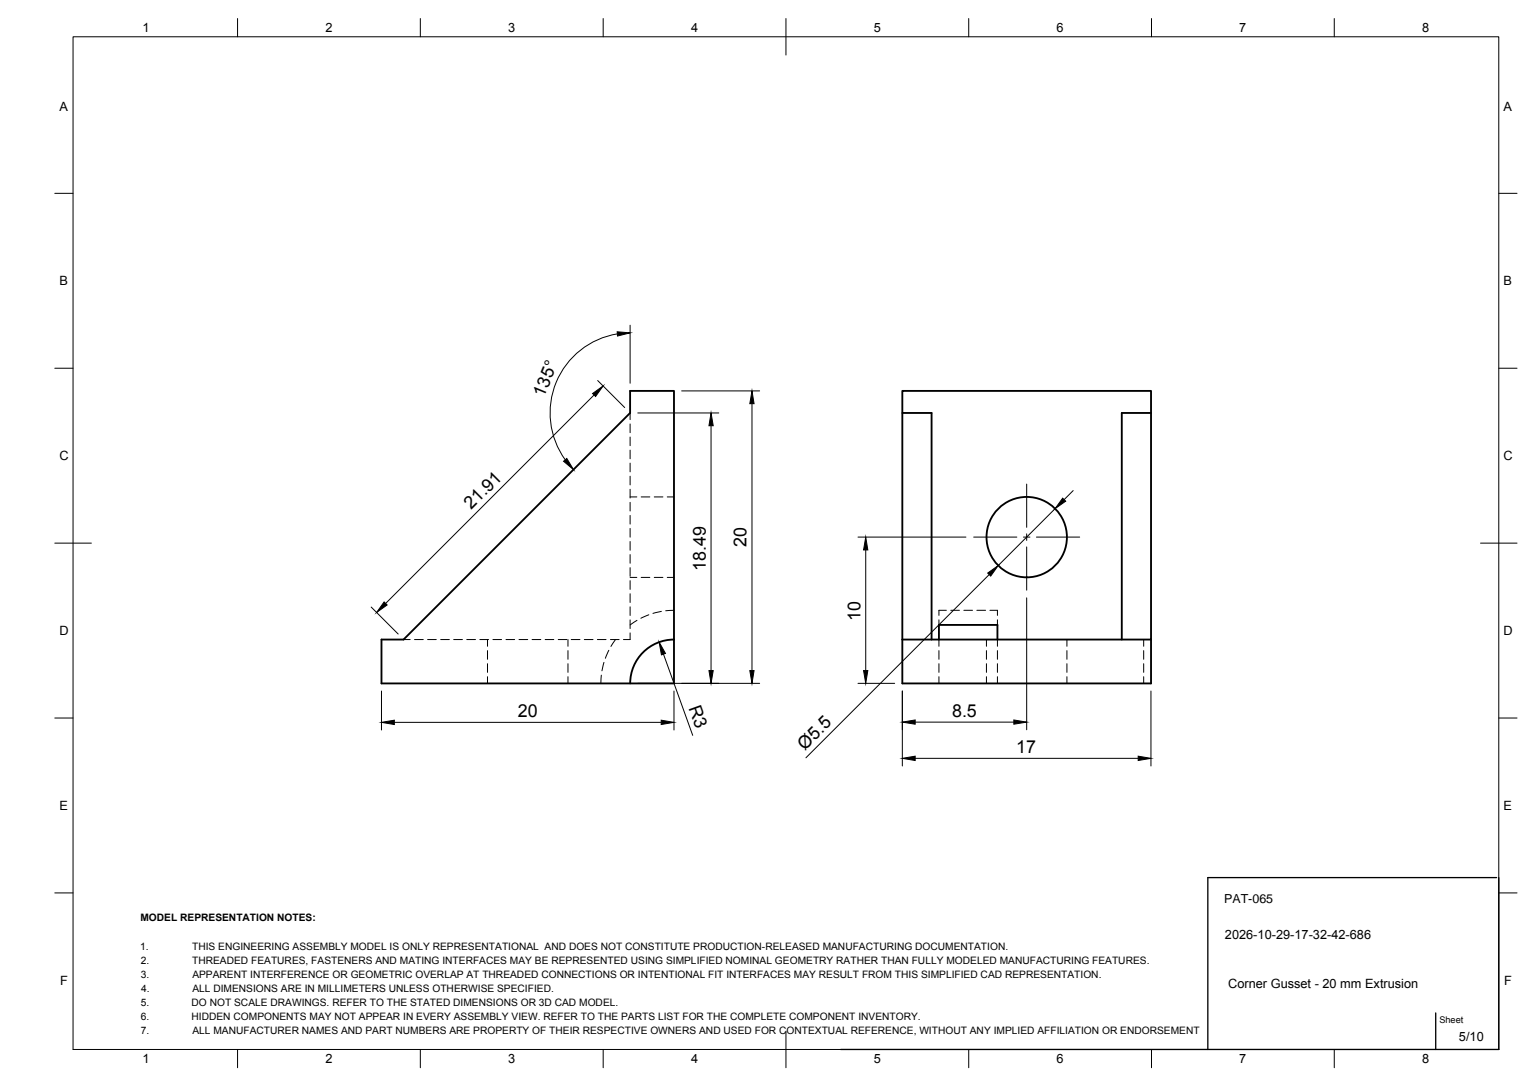
ISO-10303-21;
HEADER;
/* Generated by software containing ST-Developer
 * from STEP Tools, Inc. (www.steptools.com) 
 */

FILE_DESCRIPTION(
/* description */ ('PAT-065'),
/* implementation_level */ '2;1');

FILE_NAME(
/* name */ 'Corner Gusset - 20 mm Extrusion.step',
/* time_stamp */ '2026-10-28T22:09:22-07:00',
/* author */ (''),
/* organization */ (''),
/* preprocessor_version */ 'ST-DEVELOPER v20.2',
/* originating_system */ 'Autodesk Translation Framework v15.17.0.0',
/* authorisation */ '');

FILE_SCHEMA (('AUTOMOTIVE_DESIGN { 1 0 10303 214 3 1 1 }'));
ENDSEC;

DATA;
#10=MECHANICAL_DESIGN_GEOMETRIC_PRESENTATION_REPRESENTATION('',(#160),#5502);
#140=SHAPE_REPRESENTATION_RELATIONSHIP('SRR','None',#5557,#150);
#150=ADVANCED_BREP_SHAPE_REPRESENTATION('',(#170),#5493);
#160=STYLED_ITEM('',(#5708),#170);
#170=MANIFOLD_SOLID_BREP('Body1',#3207);
#184=FACE_BOUND('',#586,.T.);
#185=FACE_BOUND('',#588,.T.);
#186=FACE_BOUND('',#596,.T.);
#187=FACE_BOUND('',#601,.T.);
#259=PLANE('',#3412);
#260=PLANE('',#3419);
#261=PLANE('',#3420);
#262=PLANE('',#3422);
#263=PLANE('',#3424);
#264=PLANE('',#3432);
#265=PLANE('',#3433);
#266=PLANE('',#3434);
#267=PLANE('',#3435);
#268=PLANE('',#3436);
#269=PLANE('',#3437);
#270=PLANE('',#3438);
#271=PLANE('',#3439);
#272=PLANE('',#3440);
#273=PLANE('',#3441);
#400=FACE_OUTER_BOUND('',#581,.T.);
#401=FACE_OUTER_BOUND('',#582,.T.);
#402=FACE_OUTER_BOUND('',#583,.T.);
#403=FACE_OUTER_BOUND('',#584,.T.);
#404=FACE_OUTER_BOUND('',#585,.T.);
#405=FACE_OUTER_BOUND('',#587,.T.);
#406=FACE_OUTER_BOUND('',#589,.T.);
#407=FACE_OUTER_BOUND('',#590,.T.);
#408=FACE_OUTER_BOUND('',#591,.T.);
#409=FACE_OUTER_BOUND('',#592,.T.);
#410=FACE_OUTER_BOUND('',#593,.T.);
#411=FACE_OUTER_BOUND('',#594,.T.);
#412=FACE_OUTER_BOUND('',#595,.T.);
#413=FACE_OUTER_BOUND('',#597,.T.);
#414=FACE_OUTER_BOUND('',#598,.T.);
#415=FACE_OUTER_BOUND('',#599,.T.);
#416=FACE_OUTER_BOUND('',#600,.T.);
#417=FACE_OUTER_BOUND('',#602,.T.);
#418=FACE_OUTER_BOUND('',#603,.T.);
#419=FACE_OUTER_BOUND('',#604,.T.);
#581=EDGE_LOOP('',(#2512,#2513,#2514,#2515,#2516,#2517));
#582=EDGE_LOOP('',(#2518,#2519,#2520,#2521));
#583=EDGE_LOOP('',(#2522,#2523,#2524,#2525));
#584=EDGE_LOOP('',(#2526,#2527,#2528,#2529,#2530,#2531));
#585=EDGE_LOOP('',(#2532,#2533,#2534,#2535,#2536,#2537,#2538,#2539,#2540,
#2541,#2542,#2543));
#586=EDGE_LOOP('',(#2544));
#587=EDGE_LOOP('',(#2545,#2546,#2547,#2548,#2549,#2550,#2551,#2552,#2553,
#2554));
#588=EDGE_LOOP('',(#2555));
#589=EDGE_LOOP('',(#2556,#2557,#2558));
#590=EDGE_LOOP('',(#2559,#2560,#2561,#2562));
#591=EDGE_LOOP('',(#2563,#2564,#2565,#2566));
#592=EDGE_LOOP('',(#2567,#2568,#2569,#2570));
#593=EDGE_LOOP('',(#2571,#2572,#2573,#2574));
#594=EDGE_LOOP('',(#2575,#2576,#2577));
#595=EDGE_LOOP('',(#2578,#2579,#2580,#2581,#2582,#2583,#2584,#2585,#2586,
#2587,#2588,#2589));
#596=EDGE_LOOP('',(#2590));
#597=EDGE_LOOP('',(#2591,#2592,#2593,#2594));
#598=EDGE_LOOP('',(#2595,#2596,#2597));
#599=EDGE_LOOP('',(#2598,#2599,#2600,#2601,#2602,#2603,#2604,#2605));
#600=EDGE_LOOP('',(#2606,#2607,#2608,#2609,#2610,#2611,#2612,#2613,#2614,
#2615));
#601=EDGE_LOOP('',(#2616));
#602=EDGE_LOOP('',(#2617,#2618,#2619,#2620));
#603=EDGE_LOOP('',(#2621,#2622,#2623,#2624));
#604=EDGE_LOOP('',(#2625,#2626,#2627,#2628,#2629,#2630,#2631));
#870=LINE('',#4906,#1201);
#871=LINE('',#4910,#1202);
#872=LINE('',#4912,#1203);
#873=LINE('',#4915,#1204);
#874=LINE('',#4918,#1205);
#875=LINE('',#4920,#1206);
#876=LINE('',#4924,#1207);
#877=LINE('',#4927,#1208);
#878=LINE('',#4930,#1209);
#879=LINE('',#4931,#1210);
#880=LINE('',#4933,#1211);
#881=LINE('',#4934,#1212);
#882=LINE('',#4937,#1213);
#883=LINE('',#4939,#1214);
#884=LINE('',#4941,#1215);
#885=LINE('',#4943,#1216);
#886=LINE('',#4945,#1217);
#887=LINE('',#4947,#1218);
#888=LINE('',#4949,#1219);
#889=LINE('',#4951,#1220);
#890=LINE('',#4952,#1221);
#891=LINE('',#4957,#1222);
#892=LINE('',#4959,#1223);
#893=LINE('',#4961,#1224);
#894=LINE('',#4963,#1225);
#895=LINE('',#4965,#1226);
#896=LINE('',#4967,#1227);
#897=LINE('',#4968,#1228);
#898=LINE('',#4973,#1229);
#899=LINE('',#4977,#1230);
#900=LINE('',#4981,#1231);
#901=LINE('',#4986,#1232);
#902=LINE('',#4989,#1233);
#903=LINE('',#4991,#1234);
#904=LINE('',#4992,#1235);
#905=LINE('',#4994,#1236);
#906=LINE('',#4997,#1237);
#907=LINE('',#4999,#1238);
#908=LINE('',#5001,#1239);
#909=LINE('',#5003,#1240);
#910=LINE('',#5004,#1241);
#911=LINE('',#5006,#1242);
#912=LINE('',#5007,#1243);
#913=LINE('',#5011,#1244);
#914=LINE('',#5012,#1245);
#915=LINE('',#5013,#1246);
#916=LINE('',#5016,#1247);
#917=LINE('',#5017,#1248);
#918=LINE('',#5019,#1249);
#919=LINE('',#5021,#1250);
#1201=VECTOR('',#3951,1.);
#1202=VECTOR('',#3954,1.);
#1203=VECTOR('',#3955,1.);
#1204=VECTOR('',#3958,1.);
#1205=VECTOR('',#3961,1.);
#1206=VECTOR('',#3962,1.);
#1207=VECTOR('',#3967,1.);
#1208=VECTOR('',#3970,1.);
#1209=VECTOR('',#3973,1.);
#1210=VECTOR('',#3974,1.);
#1211=VECTOR('',#3975,1.);
#1212=VECTOR('',#3976,1.);
#1213=VECTOR('',#3979,1.);
#1214=VECTOR('',#3980,1.);
#1215=VECTOR('',#3981,1.);
#1216=VECTOR('',#3982,1.);
#1217=VECTOR('',#3983,1.);
#1218=VECTOR('',#3984,1.);
#1219=VECTOR('',#3985,1.);
#1220=VECTOR('',#3986,1.);
#1221=VECTOR('',#3987,1.);
#1222=VECTOR('',#3992,1.);
#1223=VECTOR('',#3993,1.);
#1224=VECTOR('',#3994,1.);
#1225=VECTOR('',#3995,1.);
#1226=VECTOR('',#3996,1.);
#1227=VECTOR('',#3997,1.);
#1228=VECTOR('',#3998,1.);
#1229=VECTOR('',#4003,1.);
#1230=VECTOR('',#4008,1.);
#1231=VECTOR('',#4013,0.275);
#1232=VECTOR('',#4020,0.275);
#1233=VECTOR('',#4023,1.);
#1234=VECTOR('',#4024,1.);
#1235=VECTOR('',#4025,1.);
#1236=VECTOR('',#4028,1.);
#1237=VECTOR('',#4031,1.);
#1238=VECTOR('',#4032,1.);
#1239=VECTOR('',#4033,1.);
#1240=VECTOR('',#4034,1.);
#1241=VECTOR('',#4035,1.);
#1242=VECTOR('',#4038,1.);
#1243=VECTOR('',#4039,1.);
#1244=VECTOR('',#4044,1.);
#1245=VECTOR('',#4045,1.);
#1246=VECTOR('',#4046,1.);
#1247=VECTOR('',#4049,1.);
#1248=VECTOR('',#4050,1.);
#1249=VECTOR('',#4053,1.);
#1250=VECTOR('',#4056,1.);
#1385=CIRCLE('',#3413,0.5);
#1386=CIRCLE('',#3414,0.5);
#1387=CIRCLE('',#3416,0.5);
#1388=CIRCLE('',#3418,0.5);
#1389=CIRCLE('',#3421,0.275);
#1390=CIRCLE('',#3423,0.275);
#1391=CIRCLE('',#3425,0.3);
#1392=CIRCLE('',#3427,0.3);
#1393=CIRCLE('',#3429,0.275);
#1394=CIRCLE('',#3431,0.275);
#1564=VERTEX_POINT('',#4904);
#1565=VERTEX_POINT('',#4905);
#1566=VERTEX_POINT('',#4907);
#1567=VERTEX_POINT('',#4909);
#1568=VERTEX_POINT('',#4911);
#1569=VERTEX_POINT('',#4913);
#1570=VERTEX_POINT('',#4917);
#1571=VERTEX_POINT('',#4919);
#1572=VERTEX_POINT('',#4923);
#1573=VERTEX_POINT('',#4925);
#1574=VERTEX_POINT('',#4929);
#1575=VERTEX_POINT('',#4932);
#1576=VERTEX_POINT('',#4936);
#1577=VERTEX_POINT('',#4938);
#1578=VERTEX_POINT('',#4940);
#1579=VERTEX_POINT('',#4942);
#1580=VERTEX_POINT('',#4944);
#1581=VERTEX_POINT('',#4946);
#1582=VERTEX_POINT('',#4948);
#1583=VERTEX_POINT('',#4950);
#1584=VERTEX_POINT('',#4953);
#1585=VERTEX_POINT('',#4956);
#1586=VERTEX_POINT('',#4958);
#1587=VERTEX_POINT('',#4960);
#1588=VERTEX_POINT('',#4962);
#1589=VERTEX_POINT('',#4964);
#1590=VERTEX_POINT('',#4966);
#1591=VERTEX_POINT('',#4969);
#1592=VERTEX_POINT('',#4972);
#1593=VERTEX_POINT('',#4976);
#1594=VERTEX_POINT('',#4980);
#1595=VERTEX_POINT('',#4984);
#1596=VERTEX_POINT('',#4988);
#1597=VERTEX_POINT('',#4990);
#1598=VERTEX_POINT('',#4996);
#1599=VERTEX_POINT('',#4998);
#1600=VERTEX_POINT('',#5000);
#1601=VERTEX_POINT('',#5002);
#1602=VERTEX_POINT('',#5010);
#1603=VERTEX_POINT('',#5015);
#1906=EDGE_CURVE('',#1564,#1565,#870,.T.);
#1907=EDGE_CURVE('',#1564,#1566,#1385,.T.);
#1908=EDGE_CURVE('',#1567,#1566,#871,.T.);
#1909=EDGE_CURVE('',#1568,#1567,#872,.T.);
#1910=EDGE_CURVE('',#1568,#1569,#1386,.T.);
#1911=EDGE_CURVE('',#1565,#1569,#873,.T.);
#1912=EDGE_CURVE('',#1569,#1570,#874,.T.);
#1913=EDGE_CURVE('',#1571,#1568,#875,.T.);
#1914=EDGE_CURVE('',#1571,#1570,#1387,.T.);
#1915=EDGE_CURVE('',#1572,#1564,#876,.T.);
#1916=EDGE_CURVE('',#1572,#1573,#1388,.T.);
#1917=EDGE_CURVE('',#1566,#1573,#877,.T.);
#1918=EDGE_CURVE('',#1574,#1572,#878,.T.);
#1919=EDGE_CURVE('',#1570,#1574,#879,.T.);
#1920=EDGE_CURVE('',#1575,#1571,#880,.T.);
#1921=EDGE_CURVE('',#1573,#1575,#881,.T.);
#1922=EDGE_CURVE('',#1576,#1565,#882,.T.);
#1923=EDGE_CURVE('',#1576,#1577,#883,.T.);
#1924=EDGE_CURVE('',#1577,#1578,#884,.T.);
#1925=EDGE_CURVE('',#1579,#1578,#885,.T.);
#1926=EDGE_CURVE('',#1579,#1580,#886,.T.);
#1927=EDGE_CURVE('',#1581,#1580,#887,.T.);
#1928=EDGE_CURVE('',#1581,#1582,#888,.T.);
#1929=EDGE_CURVE('',#1582,#1583,#889,.T.);
#1930=EDGE_CURVE('',#1574,#1583,#890,.T.);
#1931=EDGE_CURVE('',#1584,#1584,#1389,.T.);
#1932=EDGE_CURVE('',#1585,#1567,#891,.T.);
#1933=EDGE_CURVE('',#1585,#1586,#892,.T.);
#1934=EDGE_CURVE('',#1586,#1587,#893,.T.);
#1935=EDGE_CURVE('',#1588,#1587,#894,.T.);
#1936=EDGE_CURVE('',#1589,#1588,#895,.T.);
#1937=EDGE_CURVE('',#1590,#1589,#896,.T.);
#1938=EDGE_CURVE('',#1575,#1590,#897,.T.);
#1939=EDGE_CURVE('',#1591,#1591,#1390,.T.);
#1940=EDGE_CURVE('',#1592,#1585,#898,.T.);
#1941=EDGE_CURVE('',#1586,#1592,#1391,.T.);
#1942=EDGE_CURVE('',#1593,#1592,#899,.T.);
#1943=EDGE_CURVE('',#1587,#1593,#1392,.T.);
#1944=EDGE_CURVE('',#1591,#1594,#900,.T.);
#1945=EDGE_CURVE('',#1594,#1594,#1393,.T.);
#1946=EDGE_CURVE('',#1595,#1595,#1394,.T.);
#1947=EDGE_CURVE('',#1595,#1584,#901,.T.);
#1948=EDGE_CURVE('',#1596,#1581,#902,.T.);
#1949=EDGE_CURVE('',#1597,#1596,#903,.T.);
#1950=EDGE_CURVE('',#1582,#1597,#904,.T.);
#1951=EDGE_CURVE('',#1583,#1597,#905,.T.);
#1952=EDGE_CURVE('',#1598,#1596,#906,.T.);
#1953=EDGE_CURVE('',#1599,#1598,#907,.T.);
#1954=EDGE_CURVE('',#1600,#1599,#908,.T.);
#1955=EDGE_CURVE('',#1600,#1601,#909,.T.);
#1956=EDGE_CURVE('',#1601,#1576,#910,.T.);
#1957=EDGE_CURVE('',#1578,#1600,#911,.T.);
#1958=EDGE_CURVE('',#1577,#1601,#912,.T.);
#1959=EDGE_CURVE('',#1593,#1602,#913,.T.);
#1960=EDGE_CURVE('',#1602,#1579,#914,.T.);
#1961=EDGE_CURVE('',#1599,#1588,#915,.T.);
#1962=EDGE_CURVE('',#1603,#1590,#916,.T.);
#1963=EDGE_CURVE('',#1602,#1603,#917,.T.);
#1964=EDGE_CURVE('',#1580,#1603,#918,.T.);
#1965=EDGE_CURVE('',#1589,#1598,#919,.T.);
#2512=ORIENTED_EDGE('',*,*,#1906,.F.);
#2513=ORIENTED_EDGE('',*,*,#1907,.T.);
#2514=ORIENTED_EDGE('',*,*,#1908,.F.);
#2515=ORIENTED_EDGE('',*,*,#1909,.F.);
#2516=ORIENTED_EDGE('',*,*,#1910,.T.);
#2517=ORIENTED_EDGE('',*,*,#1911,.F.);
#2518=ORIENTED_EDGE('',*,*,#1912,.F.);
#2519=ORIENTED_EDGE('',*,*,#1910,.F.);
#2520=ORIENTED_EDGE('',*,*,#1913,.F.);
#2521=ORIENTED_EDGE('',*,*,#1914,.T.);
#2522=ORIENTED_EDGE('',*,*,#1915,.F.);
#2523=ORIENTED_EDGE('',*,*,#1916,.T.);
#2524=ORIENTED_EDGE('',*,*,#1917,.F.);
#2525=ORIENTED_EDGE('',*,*,#1907,.F.);
#2526=ORIENTED_EDGE('',*,*,#1918,.F.);
#2527=ORIENTED_EDGE('',*,*,#1919,.F.);
#2528=ORIENTED_EDGE('',*,*,#1914,.F.);
#2529=ORIENTED_EDGE('',*,*,#1920,.F.);
#2530=ORIENTED_EDGE('',*,*,#1921,.F.);
#2531=ORIENTED_EDGE('',*,*,#1916,.F.);
#2532=ORIENTED_EDGE('',*,*,#1918,.T.);
#2533=ORIENTED_EDGE('',*,*,#1915,.T.);
#2534=ORIENTED_EDGE('',*,*,#1906,.T.);
#2535=ORIENTED_EDGE('',*,*,#1922,.F.);
#2536=ORIENTED_EDGE('',*,*,#1923,.T.);
#2537=ORIENTED_EDGE('',*,*,#1924,.T.);
#2538=ORIENTED_EDGE('',*,*,#1925,.F.);
#2539=ORIENTED_EDGE('',*,*,#1926,.T.);
#2540=ORIENTED_EDGE('',*,*,#1927,.F.);
#2541=ORIENTED_EDGE('',*,*,#1928,.T.);
#2542=ORIENTED_EDGE('',*,*,#1929,.T.);
#2543=ORIENTED_EDGE('',*,*,#1930,.F.);
#2544=ORIENTED_EDGE('',*,*,#1931,.T.);
#2545=ORIENTED_EDGE('',*,*,#1920,.T.);
#2546=ORIENTED_EDGE('',*,*,#1913,.T.);
#2547=ORIENTED_EDGE('',*,*,#1909,.T.);
#2548=ORIENTED_EDGE('',*,*,#1932,.F.);
#2549=ORIENTED_EDGE('',*,*,#1933,.T.);
#2550=ORIENTED_EDGE('',*,*,#1934,.T.);
#2551=ORIENTED_EDGE('',*,*,#1935,.F.);
#2552=ORIENTED_EDGE('',*,*,#1936,.F.);
#2553=ORIENTED_EDGE('',*,*,#1937,.F.);
#2554=ORIENTED_EDGE('',*,*,#1938,.F.);
#2555=ORIENTED_EDGE('',*,*,#1939,.T.);
#2556=ORIENTED_EDGE('',*,*,#1940,.F.);
#2557=ORIENTED_EDGE('',*,*,#1941,.F.);
#2558=ORIENTED_EDGE('',*,*,#1933,.F.);
#2559=ORIENTED_EDGE('',*,*,#1942,.F.);
#2560=ORIENTED_EDGE('',*,*,#1943,.F.);
#2561=ORIENTED_EDGE('',*,*,#1934,.F.);
#2562=ORIENTED_EDGE('',*,*,#1941,.T.);
#2563=ORIENTED_EDGE('',*,*,#1939,.F.);
#2564=ORIENTED_EDGE('',*,*,#1944,.T.);
#2565=ORIENTED_EDGE('',*,*,#1945,.F.);
#2566=ORIENTED_EDGE('',*,*,#1944,.F.);
#2567=ORIENTED_EDGE('',*,*,#1946,.F.);
#2568=ORIENTED_EDGE('',*,*,#1947,.T.);
#2569=ORIENTED_EDGE('',*,*,#1931,.F.);
#2570=ORIENTED_EDGE('',*,*,#1947,.F.);
#2571=ORIENTED_EDGE('',*,*,#1928,.F.);
#2572=ORIENTED_EDGE('',*,*,#1948,.F.);
#2573=ORIENTED_EDGE('',*,*,#1949,.F.);
#2574=ORIENTED_EDGE('',*,*,#1950,.F.);
#2575=ORIENTED_EDGE('',*,*,#1929,.F.);
#2576=ORIENTED_EDGE('',*,*,#1950,.T.);
#2577=ORIENTED_EDGE('',*,*,#1951,.F.);
#2578=ORIENTED_EDGE('',*,*,#1919,.T.);
#2579=ORIENTED_EDGE('',*,*,#1930,.T.);
#2580=ORIENTED_EDGE('',*,*,#1951,.T.);
#2581=ORIENTED_EDGE('',*,*,#1949,.T.);
#2582=ORIENTED_EDGE('',*,*,#1952,.F.);
#2583=ORIENTED_EDGE('',*,*,#1953,.F.);
#2584=ORIENTED_EDGE('',*,*,#1954,.F.);
#2585=ORIENTED_EDGE('',*,*,#1955,.T.);
#2586=ORIENTED_EDGE('',*,*,#1956,.T.);
#2587=ORIENTED_EDGE('',*,*,#1922,.T.);
#2588=ORIENTED_EDGE('',*,*,#1911,.T.);
#2589=ORIENTED_EDGE('',*,*,#1912,.T.);
#2590=ORIENTED_EDGE('',*,*,#1945,.T.);
#2591=ORIENTED_EDGE('',*,*,#1955,.F.);
#2592=ORIENTED_EDGE('',*,*,#1957,.F.);
#2593=ORIENTED_EDGE('',*,*,#1924,.F.);
#2594=ORIENTED_EDGE('',*,*,#1958,.T.);
#2595=ORIENTED_EDGE('',*,*,#1956,.F.);
#2596=ORIENTED_EDGE('',*,*,#1958,.F.);
#2597=ORIENTED_EDGE('',*,*,#1923,.F.);
#2598=ORIENTED_EDGE('',*,*,#1943,.T.);
#2599=ORIENTED_EDGE('',*,*,#1959,.T.);
#2600=ORIENTED_EDGE('',*,*,#1960,.T.);
#2601=ORIENTED_EDGE('',*,*,#1925,.T.);
#2602=ORIENTED_EDGE('',*,*,#1957,.T.);
#2603=ORIENTED_EDGE('',*,*,#1954,.T.);
#2604=ORIENTED_EDGE('',*,*,#1961,.T.);
#2605=ORIENTED_EDGE('',*,*,#1935,.T.);
#2606=ORIENTED_EDGE('',*,*,#1921,.T.);
#2607=ORIENTED_EDGE('',*,*,#1938,.T.);
#2608=ORIENTED_EDGE('',*,*,#1962,.F.);
#2609=ORIENTED_EDGE('',*,*,#1963,.F.);
#2610=ORIENTED_EDGE('',*,*,#1959,.F.);
#2611=ORIENTED_EDGE('',*,*,#1942,.T.);
#2612=ORIENTED_EDGE('',*,*,#1940,.T.);
#2613=ORIENTED_EDGE('',*,*,#1932,.T.);
#2614=ORIENTED_EDGE('',*,*,#1908,.T.);
#2615=ORIENTED_EDGE('',*,*,#1917,.T.);
#2616=ORIENTED_EDGE('',*,*,#1946,.T.);
#2617=ORIENTED_EDGE('',*,*,#1963,.T.);
#2618=ORIENTED_EDGE('',*,*,#1964,.F.);
#2619=ORIENTED_EDGE('',*,*,#1926,.F.);
#2620=ORIENTED_EDGE('',*,*,#1960,.F.);
#2621=ORIENTED_EDGE('',*,*,#1953,.T.);
#2622=ORIENTED_EDGE('',*,*,#1965,.F.);
#2623=ORIENTED_EDGE('',*,*,#1936,.T.);
#2624=ORIENTED_EDGE('',*,*,#1961,.F.);
#2625=ORIENTED_EDGE('',*,*,#1927,.T.);
#2626=ORIENTED_EDGE('',*,*,#1964,.T.);
#2627=ORIENTED_EDGE('',*,*,#1962,.T.);
#2628=ORIENTED_EDGE('',*,*,#1937,.T.);
#2629=ORIENTED_EDGE('',*,*,#1965,.T.);
#2630=ORIENTED_EDGE('',*,*,#1952,.T.);
#2631=ORIENTED_EDGE('',*,*,#1948,.T.);
#3009=CYLINDRICAL_SURFACE('',#3415,0.5);
#3010=CYLINDRICAL_SURFACE('',#3417,0.5);
#3011=CYLINDRICAL_SURFACE('',#3426,0.3);
#3012=CYLINDRICAL_SURFACE('',#3428,0.275);
#3013=CYLINDRICAL_SURFACE('',#3430,0.275);
#3094=ADVANCED_FACE('',(#400),#259,.T.);
#3095=ADVANCED_FACE('',(#401),#3009,.F.);
#3096=ADVANCED_FACE('',(#402),#3010,.F.);
#3097=ADVANCED_FACE('',(#403),#260,.F.);
#3098=ADVANCED_FACE('',(#404,#184),#261,.T.);
#3099=ADVANCED_FACE('',(#405,#185),#262,.T.);
#3100=ADVANCED_FACE('',(#406),#263,.F.);
#3101=ADVANCED_FACE('',(#407),#3011,.F.);
#3102=ADVANCED_FACE('',(#408),#3012,.F.);
#3103=ADVANCED_FACE('',(#409),#3013,.F.);
#3104=ADVANCED_FACE('',(#410),#264,.T.);
#3105=ADVANCED_FACE('',(#411),#265,.F.);
#3106=ADVANCED_FACE('',(#412,#186),#266,.T.);
#3107=ADVANCED_FACE('',(#413),#267,.T.);
#3108=ADVANCED_FACE('',(#414),#268,.T.);
#3109=ADVANCED_FACE('',(#415),#269,.T.);
#3110=ADVANCED_FACE('',(#416,#187),#270,.T.);
#3111=ADVANCED_FACE('',(#417),#271,.T.);
#3112=ADVANCED_FACE('',(#418),#272,.T.);
#3113=ADVANCED_FACE('',(#419),#273,.T.);
#3207=CLOSED_SHELL('',(#3094,#3095,#3096,#3097,#3098,#3099,#3100,#3101,
#3102,#3103,#3104,#3105,#3106,#3107,#3108,#3109,#3110,#3111,#3112,#3113));
#3411=AXIS2_PLACEMENT_3D('',#4902,#3947,#3948);
#3412=AXIS2_PLACEMENT_3D('',#4903,#3949,#3950);
#3413=AXIS2_PLACEMENT_3D('',#4908,#3952,#3953);
#3414=AXIS2_PLACEMENT_3D('',#4914,#3956,#3957);
#3415=AXIS2_PLACEMENT_3D('',#4916,#3959,#3960);
#3416=AXIS2_PLACEMENT_3D('',#4921,#3963,#3964);
#3417=AXIS2_PLACEMENT_3D('',#4922,#3965,#3966);
#3418=AXIS2_PLACEMENT_3D('',#4926,#3968,#3969);
#3419=AXIS2_PLACEMENT_3D('',#4928,#3971,#3972);
#3420=AXIS2_PLACEMENT_3D('',#4935,#3977,#3978);
#3421=AXIS2_PLACEMENT_3D('',#4954,#3988,#3989);
#3422=AXIS2_PLACEMENT_3D('',#4955,#3990,#3991);
#3423=AXIS2_PLACEMENT_3D('',#4970,#3999,#4000);
#3424=AXIS2_PLACEMENT_3D('',#4971,#4001,#4002);
#3425=AXIS2_PLACEMENT_3D('',#4974,#4004,#4005);
#3426=AXIS2_PLACEMENT_3D('',#4975,#4006,#4007);
#3427=AXIS2_PLACEMENT_3D('',#4978,#4009,#4010);
#3428=AXIS2_PLACEMENT_3D('',#4979,#4011,#4012);
#3429=AXIS2_PLACEMENT_3D('',#4982,#4014,#4015);
#3430=AXIS2_PLACEMENT_3D('',#4983,#4016,#4017);
#3431=AXIS2_PLACEMENT_3D('',#4985,#4018,#4019);
#3432=AXIS2_PLACEMENT_3D('',#4987,#4021,#4022);
#3433=AXIS2_PLACEMENT_3D('',#4993,#4026,#4027);
#3434=AXIS2_PLACEMENT_3D('',#4995,#4029,#4030);
#3435=AXIS2_PLACEMENT_3D('',#5005,#4036,#4037);
#3436=AXIS2_PLACEMENT_3D('',#5008,#4040,#4041);
#3437=AXIS2_PLACEMENT_3D('',#5009,#4042,#4043);
#3438=AXIS2_PLACEMENT_3D('',#5014,#4047,#4048);
#3439=AXIS2_PLACEMENT_3D('',#5018,#4051,#4052);
#3440=AXIS2_PLACEMENT_3D('',#5020,#4054,#4055);
#3441=AXIS2_PLACEMENT_3D('',#5022,#4057,#4058);
#3947=DIRECTION('axis',(0.,0.,1.));
#3948=DIRECTION('refdir',(1.,0.,0.));
#3949=DIRECTION('center_axis',(0.,1.,0.));
#3950=DIRECTION('ref_axis',(1.,0.,0.));
#3951=DIRECTION('',(-1.,0.,0.));
#3952=DIRECTION('center_axis',(0.,1.,0.));
#3953=DIRECTION('ref_axis',(1.,0.,0.));
#3954=DIRECTION('',(1.,0.,0.));
#3955=DIRECTION('',(0.,0.,-1.));
#3956=DIRECTION('center_axis',(0.,1.,0.));
#3957=DIRECTION('ref_axis',(1.,0.,0.));
#3958=DIRECTION('',(0.,0.,1.));
#3959=DIRECTION('center_axis',(0.,1.,0.));
#3960=DIRECTION('ref_axis',(1.,0.,0.));
#3961=DIRECTION('',(0.,1.,0.));
#3962=DIRECTION('',(0.,-1.,0.));
#3963=DIRECTION('center_axis',(0.,1.,0.));
#3964=DIRECTION('ref_axis',(1.,0.,0.));
#3965=DIRECTION('center_axis',(0.,1.,0.));
#3966=DIRECTION('ref_axis',(1.,0.,0.));
#3967=DIRECTION('',(0.,-1.,0.));
#3968=DIRECTION('center_axis',(0.,1.,0.));
#3969=DIRECTION('ref_axis',(1.,0.,0.));
#3970=DIRECTION('',(0.,1.,0.));
#3971=DIRECTION('center_axis',(0.,1.,0.));
#3972=DIRECTION('ref_axis',(1.,0.,0.));
#3973=DIRECTION('',(1.,0.,0.));
#3974=DIRECTION('',(0.,0.,-1.));
#3975=DIRECTION('',(0.,0.,1.));
#3976=DIRECTION('',(-1.,0.,0.));
#3977=DIRECTION('center_axis',(0.,0.,1.));
#3978=DIRECTION('ref_axis',(1.,0.,0.));
#3979=DIRECTION('',(0.,1.,0.));
#3980=DIRECTION('',(1.,0.,0.));
#3981=DIRECTION('',(0.,-1.,0.));
#3982=DIRECTION('',(-1.,0.,0.));
#3983=DIRECTION('',(0.,1.,0.));
#3984=DIRECTION('',(1.,0.,0.));
#3985=DIRECTION('',(0.,-1.,0.));
#3986=DIRECTION('',(-1.,0.,0.));
#3987=DIRECTION('',(0.,1.,0.));
#3988=DIRECTION('center_axis',(0.,0.,-1.));
#3989=DIRECTION('ref_axis',(1.,0.,0.));
#3990=DIRECTION('center_axis',(-1.,0.,0.));
#3991=DIRECTION('ref_axis',(0.,0.,1.));
#3992=DIRECTION('',(0.,1.,0.));
#3993=DIRECTION('',(0.,0.,1.));
#3994=DIRECTION('',(0.,-1.,0.));
#3995=DIRECTION('',(0.,0.,-1.));
#3996=DIRECTION('',(0.,-1.,0.));
#3997=DIRECTION('',(0.,0.,1.));
#3998=DIRECTION('',(0.,1.,0.));
#3999=DIRECTION('center_axis',(1.,0.,0.));
#4000=DIRECTION('ref_axis',(0.,0.,-1.));
#4001=DIRECTION('center_axis',(0.,1.,0.));
#4002=DIRECTION('ref_axis',(1.,0.,0.));
#4003=DIRECTION('',(-1.,0.,0.));
#4004=DIRECTION('center_axis',(0.,1.,0.));
#4005=DIRECTION('ref_axis',(1.,0.,0.));
#4006=DIRECTION('center_axis',(0.,1.,0.));
#4007=DIRECTION('ref_axis',(1.,0.,0.));
#4008=DIRECTION('',(0.,1.,0.));
#4009=DIRECTION('center_axis',(0.,1.,0.));
#4010=DIRECTION('ref_axis',(1.,0.,0.));
#4011=DIRECTION('center_axis',(1.,0.,0.));
#4012=DIRECTION('ref_axis',(0.,0.,-1.));
#4013=DIRECTION('',(1.,0.,0.));
#4014=DIRECTION('center_axis',(-1.,0.,0.));
#4015=DIRECTION('ref_axis',(0.,0.,-1.));
#4016=DIRECTION('center_axis',(0.,0.,1.));
#4017=DIRECTION('ref_axis',(1.,0.,0.));
#4018=DIRECTION('center_axis',(0.,0.,1.));
#4019=DIRECTION('ref_axis',(1.,0.,0.));
#4020=DIRECTION('',(0.,0.,1.));
#4021=DIRECTION('center_axis',(0.707106781186548,0.,0.707106781186548));
#4022=DIRECTION('ref_axis',(0.707106781186548,0.,-0.707106781186548));
#4023=DIRECTION('',(0.707106781186548,0.,-0.707106781186548));
#4024=DIRECTION('',(0.,1.,0.));
#4025=DIRECTION('',(-0.707106781186548,0.,0.707106781186548));
#4026=DIRECTION('center_axis',(0.,1.,0.));
#4027=DIRECTION('ref_axis',(1.,0.,0.));
#4028=DIRECTION('',(0.,0.,1.));
#4029=DIRECTION('center_axis',(1.,0.,0.));
#4030=DIRECTION('ref_axis',(0.,0.,-1.));
#4031=DIRECTION('',(0.,0.,-1.));
#4032=DIRECTION('',(0.,1.,0.));
#4033=DIRECTION('',(0.,0.,1.));
#4034=DIRECTION('',(0.,1.,0.));
#4035=DIRECTION('',(0.,0.,-1.));
#4036=DIRECTION('center_axis',(0.707106781186548,0.,0.707106781186548));
#4037=DIRECTION('ref_axis',(-0.707106781186548,0.,0.707106781186548));
#4038=DIRECTION('',(-0.707106781186548,0.,0.707106781186548));
#4039=DIRECTION('',(-0.707106781186548,0.,0.707106781186548));
#4040=DIRECTION('center_axis',(0.,1.,0.));
#4041=DIRECTION('ref_axis',(1.,0.,0.));
#4042=DIRECTION('center_axis',(0.,-1.,0.));
#4043=DIRECTION('ref_axis',(0.,0.,-1.));
#4044=DIRECTION('',(1.,0.,0.));
#4045=DIRECTION('',(0.,0.,1.));
#4046=DIRECTION('',(-1.,0.,0.));
#4047=DIRECTION('center_axis',(0.,0.,-1.));
#4048=DIRECTION('ref_axis',(-1.,0.,0.));
#4049=DIRECTION('',(-1.,0.,0.));
#4050=DIRECTION('',(0.,1.,0.));
#4051=DIRECTION('center_axis',(1.,0.,0.));
#4052=DIRECTION('ref_axis',(0.,0.,-1.));
#4053=DIRECTION('',(0.,0.,-1.));
#4054=DIRECTION('center_axis',(0.,0.,1.));
#4055=DIRECTION('ref_axis',(1.,0.,0.));
#4056=DIRECTION('',(1.,0.,0.));
#4057=DIRECTION('center_axis',(0.,1.,0.));
#4058=DIRECTION('ref_axis',(0.,0.,1.));
#4902=CARTESIAN_POINT('',(0.,0.,0.));
#4903=CARTESIAN_POINT('Origin',(0.,0.2,0.));
#4904=CARTESIAN_POINT('',(0.4,0.2,0.3));
#4905=CARTESIAN_POINT('',(0.3,0.2,0.3));
#4906=CARTESIAN_POINT('',(0.15,0.2,0.3));
#4907=CARTESIAN_POINT('',(0.5,0.2,0.));
#4908=CARTESIAN_POINT('Origin',(0.,0.2,0.));
#4909=CARTESIAN_POINT('',(0.,0.2,0.));
#4910=CARTESIAN_POINT('',(1.,0.2,0.));
#4911=CARTESIAN_POINT('',(0.,0.2,0.5));
#4912=CARTESIAN_POINT('',(0.,0.2,0.));
#4913=CARTESIAN_POINT('',(0.3,0.2,0.4));
#4914=CARTESIAN_POINT('Origin',(0.,0.2,0.));
#4915=CARTESIAN_POINT('',(0.3,0.2,1.));
#4916=CARTESIAN_POINT('Origin',(0.,0.2,0.));
#4917=CARTESIAN_POINT('',(0.3,0.6,0.4));
#4918=CARTESIAN_POINT('',(0.3,0.2,0.4));
#4919=CARTESIAN_POINT('',(0.,0.6,0.5));
#4920=CARTESIAN_POINT('',(0.,0.2,0.5));
#4921=CARTESIAN_POINT('Origin',(0.,0.6,0.));
#4922=CARTESIAN_POINT('Origin',(0.,0.2,0.));
#4923=CARTESIAN_POINT('',(0.4,0.6,0.3));
#4924=CARTESIAN_POINT('',(0.4,0.2,0.3));
#4925=CARTESIAN_POINT('',(0.5,0.6,0.));
#4926=CARTESIAN_POINT('Origin',(0.,0.6,0.));
#4927=CARTESIAN_POINT('',(0.5,0.2,0.));
#4928=CARTESIAN_POINT('Origin',(0.,0.6,0.));
#4929=CARTESIAN_POINT('',(0.3,0.6,0.3));
#4930=CARTESIAN_POINT('',(0.15,0.6,0.3));
#4931=CARTESIAN_POINT('',(0.3,0.6,1.));
#4932=CARTESIAN_POINT('',(0.,0.6,0.));
#4933=CARTESIAN_POINT('',(0.,0.6,0.));
#4934=CARTESIAN_POINT('',(1.,0.6,0.));
#4935=CARTESIAN_POINT('Origin',(0.3,0.,0.3));
#4936=CARTESIAN_POINT('',(0.3,-0.65,0.3));
#4937=CARTESIAN_POINT('',(0.3,0.,0.3));
#4938=CARTESIAN_POINT('',(1.849,-0.65,0.3));
#4939=CARTESIAN_POINT('',(0.68725,-0.65,0.3));
#4940=CARTESIAN_POINT('',(1.849,-0.85,0.3));
#4941=CARTESIAN_POINT('',(1.849,-0.325,0.3));
#4942=CARTESIAN_POINT('',(2.,-0.85,0.3));
#4943=CARTESIAN_POINT('',(2.,-0.85,0.3));
#4944=CARTESIAN_POINT('',(2.,0.85,0.3));
#4945=CARTESIAN_POINT('',(2.,0.,0.3));
#4946=CARTESIAN_POINT('',(1.849,0.85,0.3));
#4947=CARTESIAN_POINT('',(2.,0.85,0.3));
#4948=CARTESIAN_POINT('',(1.849,0.65,0.3));
#4949=CARTESIAN_POINT('',(1.849,0.325,0.3));
#4950=CARTESIAN_POINT('',(0.3,0.65,0.3));
#4951=CARTESIAN_POINT('',(0.68725,0.65,0.3));
#4952=CARTESIAN_POINT('',(0.3,0.,0.3));
#4953=CARTESIAN_POINT('',(0.725,3.36777869765522E-17,0.3));
#4954=CARTESIAN_POINT('Origin',(1.,0.,0.3));
#4955=CARTESIAN_POINT('Origin',(0.,0.,0.));
#4956=CARTESIAN_POINT('',(0.,-0.8,0.));
#4957=CARTESIAN_POINT('',(0.,0.,0.));
#4958=CARTESIAN_POINT('',(0.,-0.8,0.3));
#4959=CARTESIAN_POINT('',(0.,-0.8,0.));
#4960=CARTESIAN_POINT('',(0.,-0.85,0.3));
#4961=CARTESIAN_POINT('',(0.,-2.1,0.3));
#4962=CARTESIAN_POINT('',(0.,-0.85,2.));
#4963=CARTESIAN_POINT('',(0.,-0.85,2.));
#4964=CARTESIAN_POINT('',(0.,0.85,2.));
#4965=CARTESIAN_POINT('',(0.,0.,2.));
#4966=CARTESIAN_POINT('',(0.,0.85,0.));
#4967=CARTESIAN_POINT('',(0.,0.85,2.));
#4968=CARTESIAN_POINT('',(0.,0.,0.));
#4969=CARTESIAN_POINT('',(0.,-3.36777869765522E-17,1.275));
#4970=CARTESIAN_POINT('Origin',(0.,0.,1.));
#4971=CARTESIAN_POINT('Origin',(0.,-0.8,0.));
#4972=CARTESIAN_POINT('',(0.3,-0.8,0.));
#4973=CARTESIAN_POINT('',(1.,-0.8,0.));
#4974=CARTESIAN_POINT('Origin',(0.,-0.8,0.));
#4975=CARTESIAN_POINT('Origin',(0.,-2.1,0.));
#4976=CARTESIAN_POINT('',(0.3,-0.85,0.));
#4977=CARTESIAN_POINT('',(0.3,-2.1,0.));
#4978=CARTESIAN_POINT('Origin',(0.,-0.85,0.));
#4979=CARTESIAN_POINT('Origin',(-0.05,0.,1.));
#4980=CARTESIAN_POINT('',(0.3,3.36777869765522E-17,1.275));
#4981=CARTESIAN_POINT('',(-0.05,-3.36777869765522E-17,1.275));
#4982=CARTESIAN_POINT('Origin',(0.3,0.,1.));
#4983=CARTESIAN_POINT('Origin',(1.,0.,-0.05));
#4984=CARTESIAN_POINT('',(0.725,-3.36777869765522E-17,0.));
#4985=CARTESIAN_POINT('Origin',(1.,0.,0.));
#4986=CARTESIAN_POINT('',(0.725,-3.36777869765522E-17,-0.05));
#4987=CARTESIAN_POINT('Origin',(0.299,0.65,1.85));
#4988=CARTESIAN_POINT('',(0.3,0.85,1.849));
#4989=CARTESIAN_POINT('',(1.85,0.85,0.299));
#4990=CARTESIAN_POINT('',(0.3,0.65,1.849));
#4991=CARTESIAN_POINT('',(0.3,0.325,1.849));
#4992=CARTESIAN_POINT('',(1.85,0.65,0.299));
#4993=CARTESIAN_POINT('Origin',(1.0745,0.65,1.0745));
#4994=CARTESIAN_POINT('',(0.3,0.65,1.53725));
#4995=CARTESIAN_POINT('Origin',(0.3,0.,2.));
#4996=CARTESIAN_POINT('',(0.3,0.85,2.));
#4997=CARTESIAN_POINT('',(0.3,0.85,0.3));
#4998=CARTESIAN_POINT('',(0.3,-0.85,2.));
#4999=CARTESIAN_POINT('',(0.3,0.,2.));
#5000=CARTESIAN_POINT('',(0.3,-0.85,1.849));
#5001=CARTESIAN_POINT('',(0.3,-0.85,0.3));
#5002=CARTESIAN_POINT('',(0.3,-0.65,1.849));
#5003=CARTESIAN_POINT('',(0.3,-0.325,1.849));
#5004=CARTESIAN_POINT('',(0.3,-0.65,1.53725));
#5005=CARTESIAN_POINT('Origin',(1.85,-0.65,0.299));
#5006=CARTESIAN_POINT('',(1.85,-0.85,0.299));
#5007=CARTESIAN_POINT('',(1.85,-0.65,0.299));
#5008=CARTESIAN_POINT('Origin',(1.0745,-0.65,1.0745));
#5009=CARTESIAN_POINT('Origin',(1.,-0.85,1.));
#5010=CARTESIAN_POINT('',(2.,-0.85,0.));
#5011=CARTESIAN_POINT('',(0.,-0.85,0.));
#5012=CARTESIAN_POINT('',(2.,-0.85,0.));
#5013=CARTESIAN_POINT('',(0.3,-0.85,2.));
#5014=CARTESIAN_POINT('Origin',(2.,0.,0.));
#5015=CARTESIAN_POINT('',(2.,0.85,0.));
#5016=CARTESIAN_POINT('',(0.,0.85,0.));
#5017=CARTESIAN_POINT('',(2.,0.,0.));
#5018=CARTESIAN_POINT('Origin',(2.,0.,0.3));
#5019=CARTESIAN_POINT('',(2.,0.85,0.));
#5020=CARTESIAN_POINT('Origin',(0.,0.,2.));
#5021=CARTESIAN_POINT('',(0.3,0.85,2.));
#5022=CARTESIAN_POINT('Origin',(1.,0.85,1.));
#5480=UNCERTAINTY_MEASURE_WITH_UNIT(LENGTH_MEASURE(0.001),#5503,
'DISTANCE_ACCURACY_VALUE',
'Maximum model space distance between geometric entities at asserted c
onnectivities');
#5489=UNCERTAINTY_MEASURE_WITH_UNIT(LENGTH_MEASURE(0.001),#5503,
'DISTANCE_ACCURACY_VALUE',
'Maximum model space distance between geometric entities at asserted c
onnectivities');
#5493=(
GEOMETRIC_REPRESENTATION_CONTEXT(3)
GLOBAL_UNCERTAINTY_ASSIGNED_CONTEXT((#5480))
GLOBAL_UNIT_ASSIGNED_CONTEXT((#5503,#5505,#5506))
REPRESENTATION_CONTEXT('','3D')
);
#5502=(
GEOMETRIC_REPRESENTATION_CONTEXT(3)
GLOBAL_UNCERTAINTY_ASSIGNED_CONTEXT((#5489))
GLOBAL_UNIT_ASSIGNED_CONTEXT((#5503,#5505,#5506))
REPRESENTATION_CONTEXT('','3D')
);
#5503=(
LENGTH_UNIT()
NAMED_UNIT(*)
SI_UNIT(.CENTI.,.METRE.)
);
#5505=(
NAMED_UNIT(*)
PLANE_ANGLE_UNIT()
SI_UNIT($,.RADIAN.)
);
#5506=(
NAMED_UNIT(*)
SI_UNIT($,.STERADIAN.)
SOLID_ANGLE_UNIT()
);
#5510=SHAPE_DEFINITION_REPRESENTATION(#5522,#5557);
#5522=PRODUCT_DEFINITION_SHAPE('',$,#5570);
#5557=SHAPE_REPRESENTATION('',(#3411),#5493);
#5566=PRODUCT_DEFINITION_CONTEXT('part definition',#5604,'design');
#5570=PRODUCT_DEFINITION('Corner Gusset - 20 mm Extrusion',
'Corner Gusset - 20 mm Extrusion',#5582,#5566);
#5582=PRODUCT_DEFINITION_FORMATION('',$,#5609);
#5604=APPLICATION_CONTEXT(
'Core Data for Automotive Mechanical Design Process');
#5605=PRODUCT_CONTEXT('part definition',#5604,'mechanical');
#5609=PRODUCT('Corner Gusset - 20 mm Extrusion',
'Corner Gusset - 20 mm Extrusion','Corner Gusset - 20 mm Extrusion',(#5605));
#5702=COLOUR_RGB('Off White',0.89,0.88,0.83);
#5703=FILL_AREA_STYLE_COLOUR('',#5702);
#5704=FILL_AREA_STYLE('',(#5703));
#5705=SURFACE_STYLE_FILL_AREA(#5704);
#5706=SURFACE_SIDE_STYLE('',(#5705));
#5707=SURFACE_STYLE_USAGE(.BOTH.,#5706);
#5708=PRESENTATION_STYLE_ASSIGNMENT((#5707));
ENDSEC;
END-ISO-10303-21;
